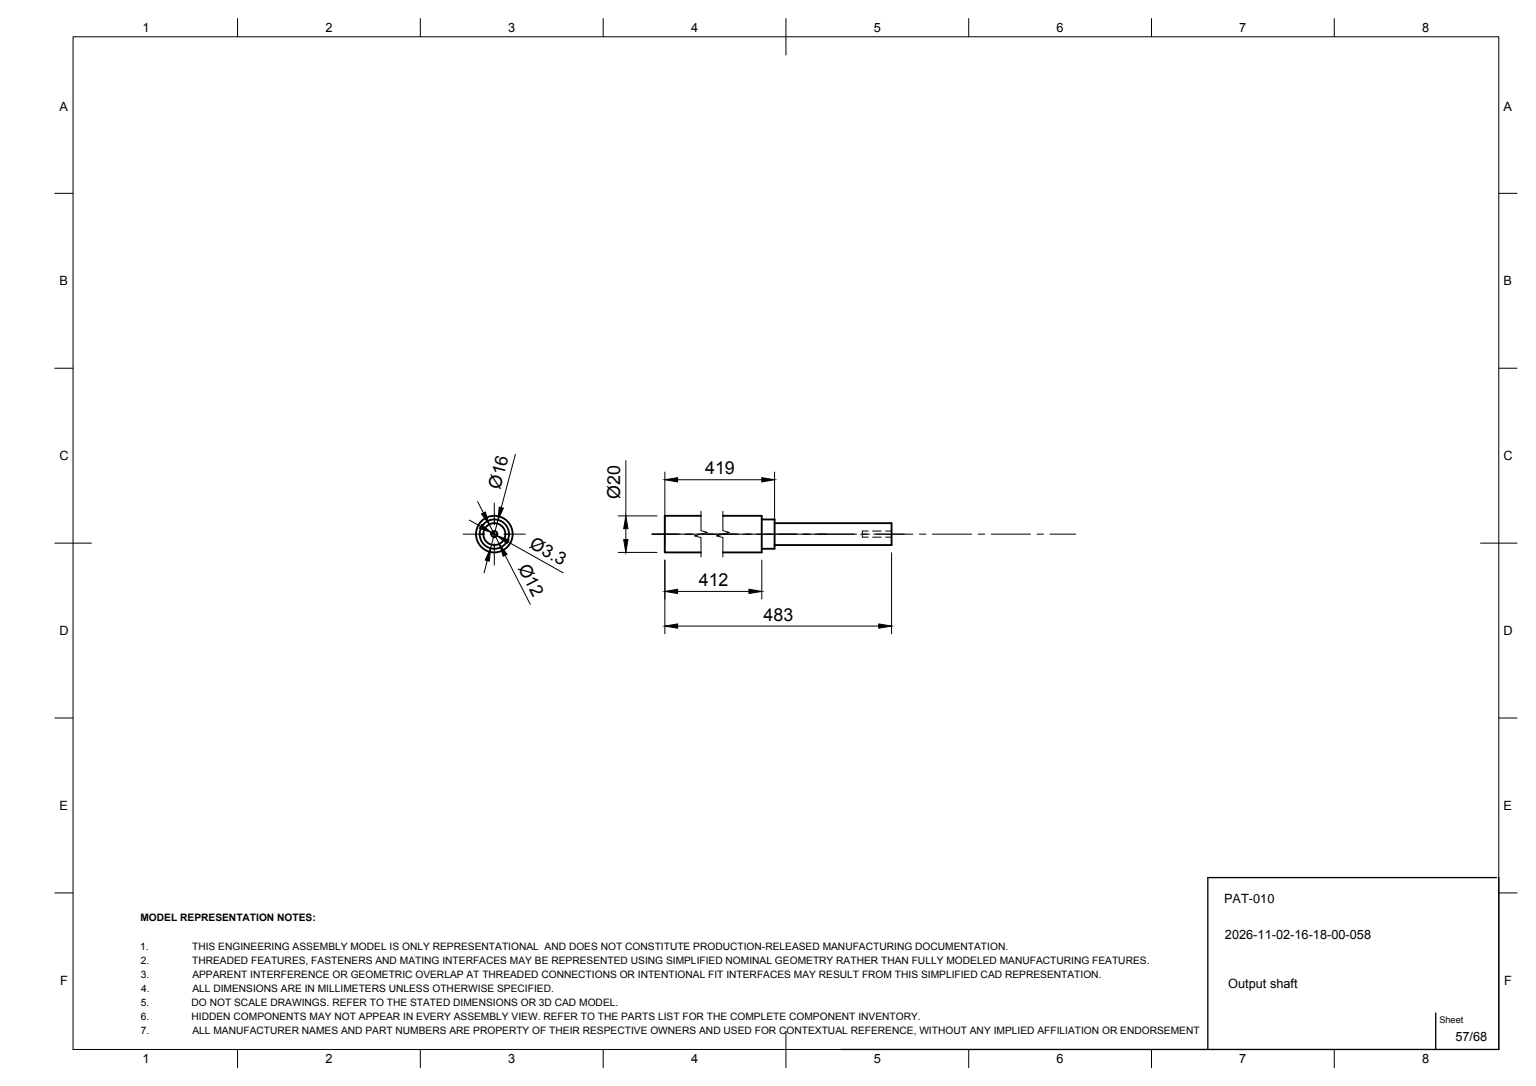
ISO-10303-21;
HEADER;
/* Generated by software containing ST-Developer
 * from STEP Tools, Inc. (www.steptools.com) 
 */

FILE_DESCRIPTION(
/* description */ ('Belt conveyor head drive unit'),
/* implementation_level */ '2;1');

FILE_NAME(
/* name */ 'Output shaft.step',
/* time_stamp */ '2026-10-28T03:26:19-07:00',
/* author */ (''),
/* organization */ (''),
/* preprocessor_version */ 'ST-DEVELOPER v20.2',
/* originating_system */ 'Autodesk Translation Framework v15.17.0.0',
/* authorisation */ '');

FILE_SCHEMA (('AUTOMOTIVE_DESIGN { 1 0 10303 214 3 1 1 }'));
ENDSEC;

DATA;
#10=MECHANICAL_DESIGN_GEOMETRIC_PRESENTATION_REPRESENTATION('',(#916),#27069);
#762=SHAPE_REPRESENTATION_RELATIONSHIP('SRR','None',#27411,#831);
#831=ADVANCED_BREP_SHAPE_REPRESENTATION('',(#997),#27053);
#916=STYLED_ITEM('',(#27797),#997);
#997=MANIFOLD_SOLID_BREP('Body1',#13785);
#1233=FACE_BOUND('',#3266,.T.);
#1234=FACE_BOUND('',#3272,.T.);
#1235=FACE_BOUND('',#3276,.T.);
#1571=PLANE('',#15873);
#1572=PLANE('',#15878);
#1573=PLANE('',#15882);
#1574=PLANE('',#15883);
#1575=PLANE('',#15889);
#2244=FACE_OUTER_BOUND('',#3265,.T.);
#2245=FACE_OUTER_BOUND('',#3267,.T.);
#2246=FACE_OUTER_BOUND('',#3268,.T.);
#2247=FACE_OUTER_BOUND('',#3269,.T.);
#2248=FACE_OUTER_BOUND('',#3270,.T.);
#2249=FACE_OUTER_BOUND('',#3271,.T.);
#2250=FACE_OUTER_BOUND('',#3273,.T.);
#2251=FACE_OUTER_BOUND('',#3274,.T.);
#2252=FACE_OUTER_BOUND('',#3275,.T.);
#3265=EDGE_LOOP('',(#11622));
#3266=EDGE_LOOP('',(#11623));
#3267=EDGE_LOOP('',(#11624,#11625,#11626,#11627));
#3268=EDGE_LOOP('',(#11628));
#3269=EDGE_LOOP('',(#11629,#11630,#11631,#11632));
#3270=EDGE_LOOP('',(#11633));
#3271=EDGE_LOOP('',(#11634));
#3272=EDGE_LOOP('',(#11635));
#3273=EDGE_LOOP('',(#11636,#11637,#11638,#11639));
#3274=EDGE_LOOP('',(#11640,#11641,#11642,#11643));
#3275=EDGE_LOOP('',(#11644));
#3276=EDGE_LOOP('',(#11645));
#4117=LINE('',#25328,#4909);
#4118=LINE('',#25334,#4910);
#4119=LINE('',#25343,#4911);
#4120=LINE('',#25346,#4912);
#4909=VECTOR('',#19685,1.);
#4910=VECTOR('',#19692,0.165);
#4911=VECTOR('',#19705,0.8);
#4912=VECTOR('',#19708,0.6);
#5709=CIRCLE('',#15874,1.);
#5710=CIRCLE('',#15875,0.8);
#5711=CIRCLE('',#15877,1.);
#5712=CIRCLE('',#15880,0.165);
#5713=CIRCLE('',#15881,0.165);
#5714=CIRCLE('',#15884,0.8);
#5715=CIRCLE('',#15885,0.6);
#5716=CIRCLE('',#15888,0.6);
#6865=VERTEX_POINT('',#25321);
#6866=VERTEX_POINT('',#25323);
#6867=VERTEX_POINT('',#25326);
#6868=VERTEX_POINT('',#25331);
#6869=VERTEX_POINT('',#25333);
#6870=VERTEX_POINT('',#25338);
#6871=VERTEX_POINT('',#25340);
#6872=VERTEX_POINT('',#25345);
#8503=EDGE_CURVE('',#6865,#6865,#5709,.T.);
#8504=EDGE_CURVE('',#6866,#6866,#5710,.T.);
#8505=EDGE_CURVE('',#6867,#6867,#5711,.T.);
#8506=EDGE_CURVE('',#6867,#6865,#4117,.T.);
#8507=EDGE_CURVE('',#6868,#6868,#5712,.T.);
#8508=EDGE_CURVE('',#6868,#6869,#4118,.T.);
#8509=EDGE_CURVE('',#6869,#6869,#5713,.T.);
#8510=EDGE_CURVE('',#6870,#6870,#5714,.T.);
#8511=EDGE_CURVE('',#6871,#6871,#5715,.T.);
#8512=EDGE_CURVE('',#6866,#6870,#4119,.T.);
#8513=EDGE_CURVE('',#6871,#6872,#4120,.T.);
#8514=EDGE_CURVE('',#6872,#6872,#5716,.T.);
#11622=ORIENTED_EDGE('',*,*,#8503,.F.);
#11623=ORIENTED_EDGE('',*,*,#8504,.T.);
#11624=ORIENTED_EDGE('',*,*,#8505,.F.);
#11625=ORIENTED_EDGE('',*,*,#8506,.T.);
#11626=ORIENTED_EDGE('',*,*,#8503,.T.);
#11627=ORIENTED_EDGE('',*,*,#8506,.F.);
#11628=ORIENTED_EDGE('',*,*,#8505,.T.);
#11629=ORIENTED_EDGE('',*,*,#8507,.F.);
#11630=ORIENTED_EDGE('',*,*,#8508,.T.);
#11631=ORIENTED_EDGE('',*,*,#8509,.T.);
#11632=ORIENTED_EDGE('',*,*,#8508,.F.);
#11633=ORIENTED_EDGE('',*,*,#8509,.F.);
#11634=ORIENTED_EDGE('',*,*,#8510,.F.);
#11635=ORIENTED_EDGE('',*,*,#8511,.F.);
#11636=ORIENTED_EDGE('',*,*,#8504,.F.);
#11637=ORIENTED_EDGE('',*,*,#8512,.T.);
#11638=ORIENTED_EDGE('',*,*,#8510,.T.);
#11639=ORIENTED_EDGE('',*,*,#8512,.F.);
#11640=ORIENTED_EDGE('',*,*,#8511,.T.);
#11641=ORIENTED_EDGE('',*,*,#8513,.T.);
#11642=ORIENTED_EDGE('',*,*,#8514,.T.);
#11643=ORIENTED_EDGE('',*,*,#8513,.F.);
#11644=ORIENTED_EDGE('',*,*,#8514,.F.);
#11645=ORIENTED_EDGE('',*,*,#8507,.T.);
#12791=CYLINDRICAL_SURFACE('',#15876,1.);
#12792=CYLINDRICAL_SURFACE('',#15879,0.165);
#12793=CYLINDRICAL_SURFACE('',#15886,0.8);
#12794=CYLINDRICAL_SURFACE('',#15887,0.6);
#13523=ADVANCED_FACE('',(#2244,#1233),#1571,.F.);
#13524=ADVANCED_FACE('',(#2245),#12791,.T.);
#13525=ADVANCED_FACE('',(#2246),#1572,.T.);
#13526=ADVANCED_FACE('',(#2247),#12792,.F.);
#13527=ADVANCED_FACE('',(#2248),#1573,.F.);
#13528=ADVANCED_FACE('',(#2249,#1234),#1574,.F.);
#13529=ADVANCED_FACE('',(#2250),#12793,.T.);
#13530=ADVANCED_FACE('',(#2251),#12794,.T.);
#13531=ADVANCED_FACE('',(#2252,#1235),#1575,.F.);
#13785=CLOSED_SHELL('',(#13523,#13524,#13525,#13526,#13527,#13528,#13529,
#13530,#13531));
#15872=AXIS2_PLACEMENT_3D('',#25319,#19673,#19674);
#15873=AXIS2_PLACEMENT_3D('',#25320,#19675,#19676);
#15874=AXIS2_PLACEMENT_3D('',#25322,#19677,#19678);
#15875=AXIS2_PLACEMENT_3D('',#25324,#19679,#19680);
#15876=AXIS2_PLACEMENT_3D('',#25325,#19681,#19682);
#15877=AXIS2_PLACEMENT_3D('',#25327,#19683,#19684);
#15878=AXIS2_PLACEMENT_3D('',#25329,#19686,#19687);
#15879=AXIS2_PLACEMENT_3D('',#25330,#19688,#19689);
#15880=AXIS2_PLACEMENT_3D('',#25332,#19690,#19691);
#15881=AXIS2_PLACEMENT_3D('',#25335,#19693,#19694);
#15882=AXIS2_PLACEMENT_3D('',#25336,#19695,#19696);
#15883=AXIS2_PLACEMENT_3D('',#25337,#19697,#19698);
#15884=AXIS2_PLACEMENT_3D('',#25339,#19699,#19700);
#15885=AXIS2_PLACEMENT_3D('',#25341,#19701,#19702);
#15886=AXIS2_PLACEMENT_3D('',#25342,#19703,#19704);
#15887=AXIS2_PLACEMENT_3D('',#25344,#19706,#19707);
#15888=AXIS2_PLACEMENT_3D('',#25347,#19709,#19710);
#15889=AXIS2_PLACEMENT_3D('',#25348,#19711,#19712);
#19673=DIRECTION('axis',(0.,0.,1.));
#19674=DIRECTION('refdir',(1.,0.,0.));
#19675=DIRECTION('center_axis',(0.,1.,0.));
#19676=DIRECTION('ref_axis',(1.,0.,0.));
#19677=DIRECTION('center_axis',(0.,1.,0.));
#19678=DIRECTION('ref_axis',(1.,0.,0.));
#19679=DIRECTION('center_axis',(0.,1.,0.));
#19680=DIRECTION('ref_axis',(1.,0.,0.));
#19681=DIRECTION('center_axis',(0.,1.,0.));
#19682=DIRECTION('ref_axis',(1.,0.,0.));
#19683=DIRECTION('center_axis',(0.,1.,0.));
#19684=DIRECTION('ref_axis',(1.,0.,0.));
#19685=DIRECTION('',(0.,-1.,0.));
#19686=DIRECTION('center_axis',(0.,1.,0.));
#19687=DIRECTION('ref_axis',(1.,0.,0.));
#19688=DIRECTION('center_axis',(0.,1.,0.));
#19689=DIRECTION('ref_axis',(1.,0.,0.));
#19690=DIRECTION('center_axis',(0.,1.,0.));
#19691=DIRECTION('ref_axis',(1.,0.,0.));
#19692=DIRECTION('',(0.,1.,0.));
#19693=DIRECTION('center_axis',(0.,1.,0.));
#19694=DIRECTION('ref_axis',(1.,0.,0.));
#19695=DIRECTION('center_axis',(0.,1.,0.));
#19696=DIRECTION('ref_axis',(1.,0.,0.));
#19697=DIRECTION('center_axis',(0.,1.,0.));
#19698=DIRECTION('ref_axis',(1.,0.,0.));
#19699=DIRECTION('center_axis',(0.,1.,0.));
#19700=DIRECTION('ref_axis',(1.,0.,0.));
#19701=DIRECTION('center_axis',(0.,-1.,0.));
#19702=DIRECTION('ref_axis',(1.,0.,0.));
#19703=DIRECTION('center_axis',(0.,1.,0.));
#19704=DIRECTION('ref_axis',(1.,0.,0.));
#19705=DIRECTION('',(0.,-1.,0.));
#19706=DIRECTION('center_axis',(0.,1.,0.));
#19707=DIRECTION('ref_axis',(1.,0.,0.));
#19708=DIRECTION('',(0.,-1.,0.));
#19709=DIRECTION('center_axis',(0.,1.,0.));
#19710=DIRECTION('ref_axis',(1.,0.,0.));
#19711=DIRECTION('center_axis',(0.,1.,0.));
#19712=DIRECTION('ref_axis',(1.,0.,0.));
#25319=CARTESIAN_POINT('',(0.,0.,0.));
#25320=CARTESIAN_POINT('Origin',(6.97091003018116,2.1,7.));
#25321=CARTESIAN_POINT('',(5.97091003018116,2.1,7.));
#25322=CARTESIAN_POINT('Origin',(6.97091003018116,2.1,7.));
#25323=CARTESIAN_POINT('',(6.17091003018116,2.1,7.));
#25324=CARTESIAN_POINT('Origin',(6.97091003018116,2.1,7.));
#25325=CARTESIAN_POINT('Origin',(6.97091003018116,2.1,7.));
#25326=CARTESIAN_POINT('',(5.97091003018116,43.3,7.));
#25327=CARTESIAN_POINT('Origin',(6.97091003018116,43.3,7.));
#25328=CARTESIAN_POINT('',(5.97091003018116,2.1,7.));
#25329=CARTESIAN_POINT('Origin',(6.97091003018116,43.3,7.));
#25330=CARTESIAN_POINT('Origin',(6.97091003018116,-5.1,7.));
#25331=CARTESIAN_POINT('',(6.80591003018116,-5.,7.));
#25332=CARTESIAN_POINT('Origin',(6.97091003018116,-5.,7.));
#25333=CARTESIAN_POINT('',(6.80591003018116,-3.4,7.));
#25334=CARTESIAN_POINT('',(6.80591003018116,-5.1,7.));
#25335=CARTESIAN_POINT('Origin',(6.97091003018116,-3.4,7.));
#25336=CARTESIAN_POINT('Origin',(6.97091003018116,-3.4,7.));
#25337=CARTESIAN_POINT('Origin',(6.97091003018116,1.4,7.));
#25338=CARTESIAN_POINT('',(6.17091003018116,1.4,7.));
#25339=CARTESIAN_POINT('Origin',(6.97091003018116,1.4,7.));
#25340=CARTESIAN_POINT('',(6.37091003018116,1.4,7.));
#25341=CARTESIAN_POINT('Origin',(6.97091003018116,1.4,7.));
#25342=CARTESIAN_POINT('Origin',(6.97091003018116,1.4,7.));
#25343=CARTESIAN_POINT('',(6.17091003018116,1.4,7.));
#25344=CARTESIAN_POINT('Origin',(6.97091003018116,-1.8,7.));
#25345=CARTESIAN_POINT('',(6.37091003018116,-5.,7.));
#25346=CARTESIAN_POINT('',(6.37091003018116,-1.8,7.));
#25347=CARTESIAN_POINT('Origin',(6.97091003018116,-5.,7.));
#25348=CARTESIAN_POINT('Origin',(6.97091003018116,-5.,7.));
#26976=UNCERTAINTY_MEASURE_WITH_UNIT(LENGTH_MEASURE(0.001),#27070,
'DISTANCE_ACCURACY_VALUE',
'Maximum model space distance between geometric entities at asserted c
onnectivities');
#26992=UNCERTAINTY_MEASURE_WITH_UNIT(LENGTH_MEASURE(0.001),#27070,
'DISTANCE_ACCURACY_VALUE',
'Maximum model space distance between geometric entities at asserted c
onnectivities');
#27053=(
GEOMETRIC_REPRESENTATION_CONTEXT(3)
GLOBAL_UNCERTAINTY_ASSIGNED_CONTEXT((#26976))
GLOBAL_UNIT_ASSIGNED_CONTEXT((#27070,#27072,#27073))
REPRESENTATION_CONTEXT('','3D')
);
#27069=(
GEOMETRIC_REPRESENTATION_CONTEXT(3)
GLOBAL_UNCERTAINTY_ASSIGNED_CONTEXT((#26992))
GLOBAL_UNIT_ASSIGNED_CONTEXT((#27070,#27072,#27073))
REPRESENTATION_CONTEXT('','3D')
);
#27070=(
LENGTH_UNIT()
NAMED_UNIT(*)
SI_UNIT(.CENTI.,.METRE.)
);
#27072=(
NAMED_UNIT(*)
PLANE_ANGLE_UNIT()
SI_UNIT($,.RADIAN.)
);
#27073=(
NAMED_UNIT(*)
SI_UNIT($,.STERADIAN.)
SOLID_ANGLE_UNIT()
);
#27134=SHAPE_DEFINITION_REPRESENTATION(#27222,#27411);
#27222=PRODUCT_DEFINITION_SHAPE('',$,#27488);
#27411=SHAPE_REPRESENTATION('',(#15872),#27053);
#27427=PRODUCT_DEFINITION_CONTEXT('part definition',#27657,'design');
#27488=PRODUCT_DEFINITION('Output shaft','Output shaft',#27564,#27427);
#27564=PRODUCT_DEFINITION_FORMATION('',$,#27719);
#27657=APPLICATION_CONTEXT(
'Core Data for Automotive Mechanical Design Process');
#27658=PRODUCT_CONTEXT('part definition',#27657,'mechanical');
#27719=PRODUCT('Output shaft','Output shaft','Output shaft',(#27658));
#27791=COLOUR_RGB('Grey',0.48,0.52,0.57);
#27792=FILL_AREA_STYLE_COLOUR('',#27791);
#27793=FILL_AREA_STYLE('',(#27792));
#27794=SURFACE_STYLE_FILL_AREA(#27793);
#27795=SURFACE_SIDE_STYLE('',(#27794));
#27796=SURFACE_STYLE_USAGE(.BOTH.,#27795);
#27797=PRESENTATION_STYLE_ASSIGNMENT((#27796));
ENDSEC;
END-ISO-10303-21;
